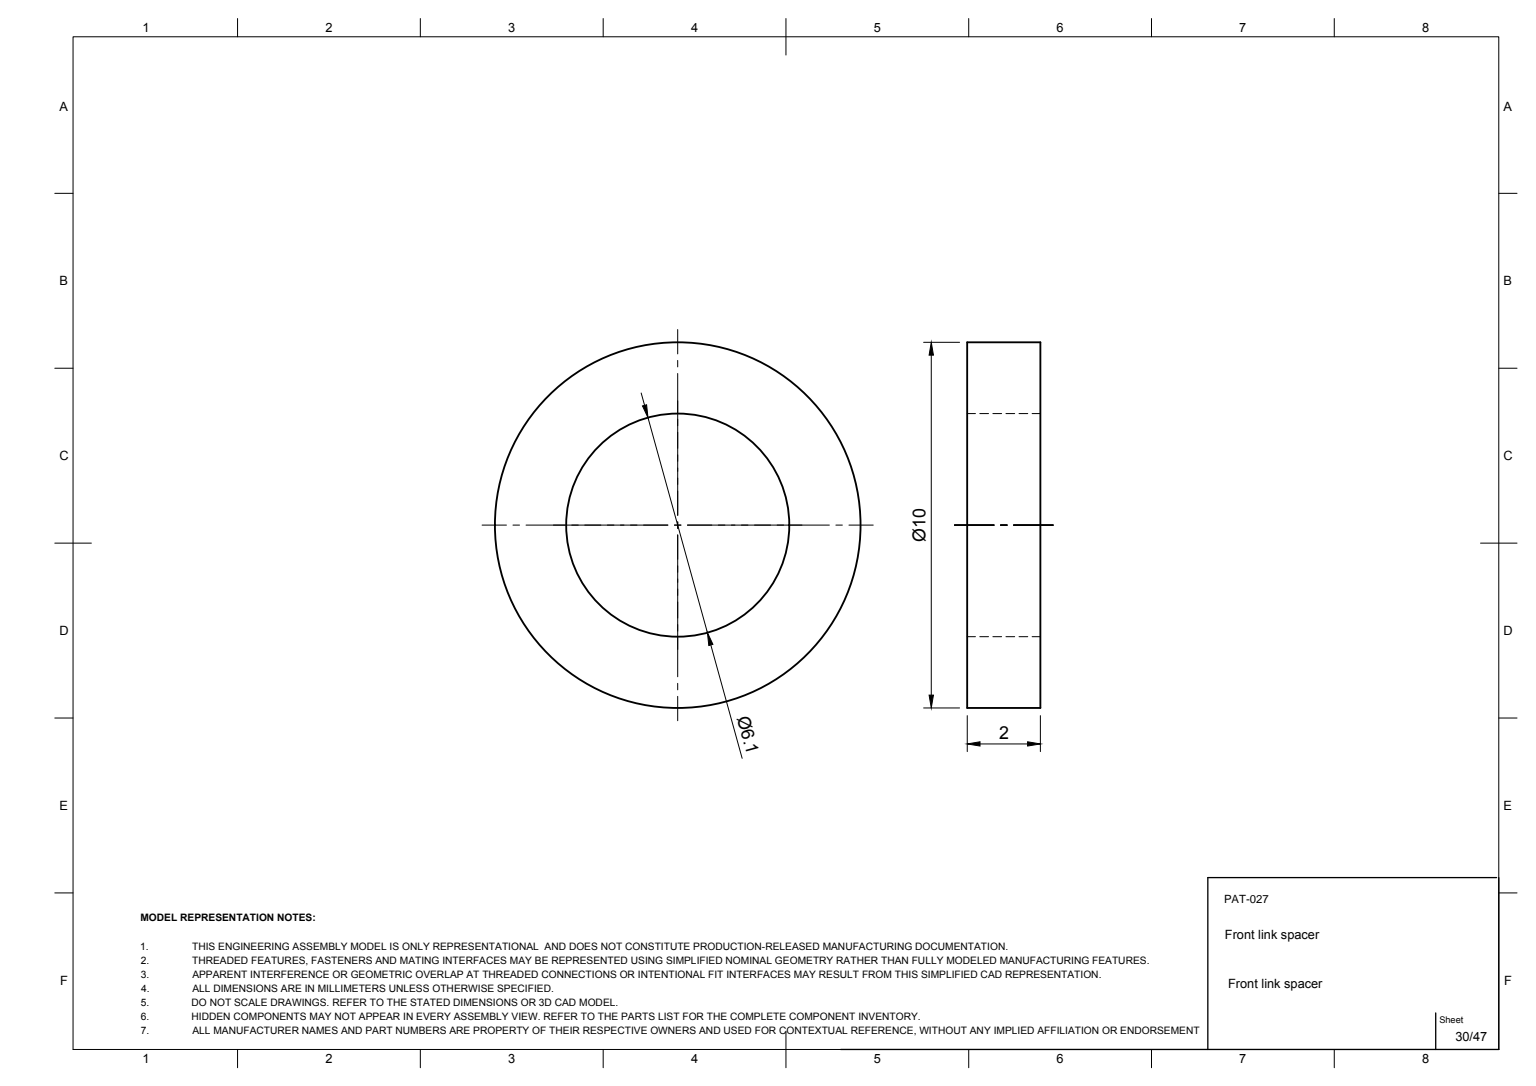
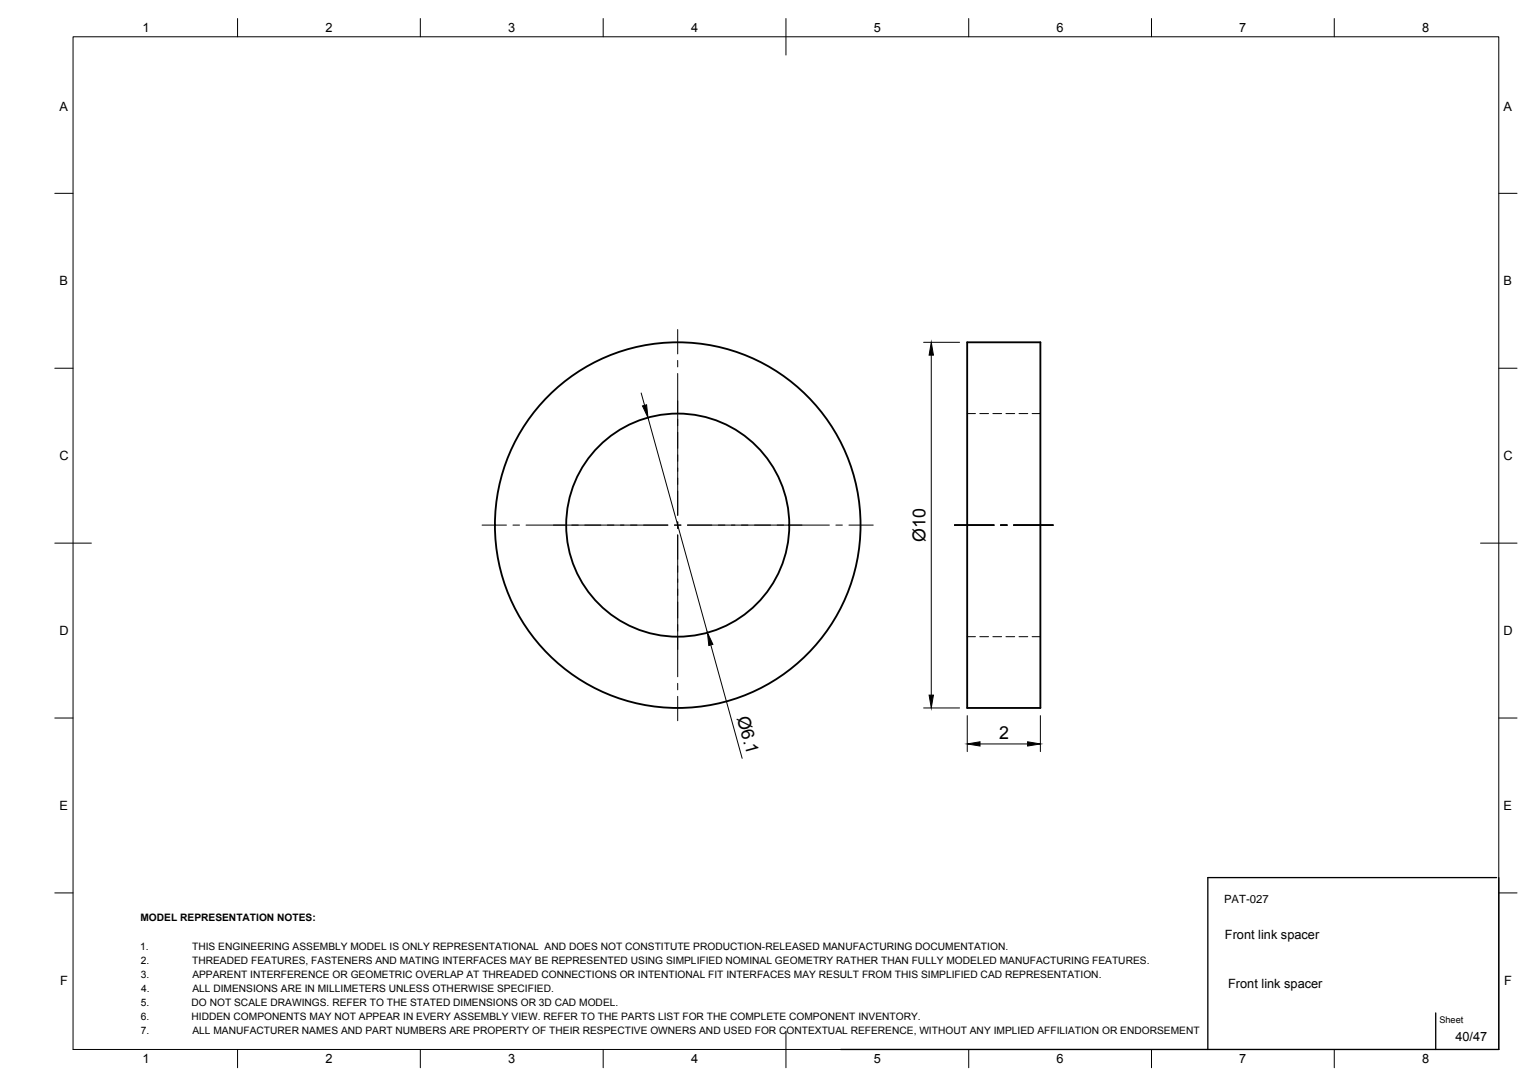
ISO-10303-21;
HEADER;
/* Generated by software containing ST-Developer
 * from STEP Tools, Inc. (www.steptools.com) 
 */

FILE_DESCRIPTION(
/* description */ ('Crank-driven oscillating fan base (mechanism only)'),

/* implementation_level */ '2;1');

FILE_NAME(
/* name */ 'Front link spacer.step',
/* time_stamp */ '2026-10-28T03:25:00-07:00',
/* author */ (''),
/* organization */ (''),
/* preprocessor_version */ 'ST-DEVELOPER v20.2',
/* originating_system */ 'Autodesk Translation Framework v15.17.0.0',
/* authorisation */ '');

FILE_SCHEMA (('AUTOMOTIVE_DESIGN { 1 0 10303 214 3 1 1 }'));
ENDSEC;

DATA;
#10=MECHANICAL_DESIGN_GEOMETRIC_PRESENTATION_REPRESENTATION('',(#467),#11916);
#379=SHAPE_REPRESENTATION_RELATIONSHIP('SRR','None',#12105,#419);
#419=ADVANCED_BREP_SHAPE_REPRESENTATION('',(#514),#11896);
#467=STYLED_ITEM('',(#12361),#514);
#514=MANIFOLD_SOLID_BREP('Body1',#6098);
#642=FACE_BOUND('',#1607,.T.);
#643=FACE_BOUND('',#1609,.T.);
#800=PLANE('',#7087);
#801=PLANE('',#7088);
#1117=FACE_OUTER_BOUND('',#1604,.T.);
#1118=FACE_OUTER_BOUND('',#1605,.T.);
#1119=FACE_OUTER_BOUND('',#1606,.T.);
#1120=FACE_OUTER_BOUND('',#1608,.T.);
#1604=EDGE_LOOP('',(#5012,#5013,#5014,#5015));
#1605=EDGE_LOOP('',(#5016,#5017,#5018,#5019));
#1606=EDGE_LOOP('',(#5020));
#1607=EDGE_LOOP('',(#5021));
#1608=EDGE_LOOP('',(#5022));
#1609=EDGE_LOOP('',(#5023));
#1975=LINE('',#11100,#2308);
#1976=LINE('',#11106,#2309);
#2308=VECTOR('',#8636,0.305);
#2309=VECTOR('',#8643,0.5);
#2723=CIRCLE('',#7082,0.305);
#2724=CIRCLE('',#7083,0.305);
#2725=CIRCLE('',#7085,0.5);
#2726=CIRCLE('',#7086,0.5);
#3154=VERTEX_POINT('',#11097);
#3155=VERTEX_POINT('',#11099);
#3156=VERTEX_POINT('',#11103);
#3157=VERTEX_POINT('',#11105);
#3801=EDGE_CURVE('',#3154,#3154,#2723,.T.);
#3802=EDGE_CURVE('',#3154,#3155,#1975,.T.);
#3803=EDGE_CURVE('',#3155,#3155,#2724,.T.);
#3804=EDGE_CURVE('',#3156,#3156,#2725,.T.);
#3805=EDGE_CURVE('',#3156,#3157,#1976,.T.);
#3806=EDGE_CURVE('',#3157,#3157,#2726,.T.);
#5012=ORIENTED_EDGE('',*,*,#3801,.F.);
#5013=ORIENTED_EDGE('',*,*,#3802,.T.);
#5014=ORIENTED_EDGE('',*,*,#3803,.T.);
#5015=ORIENTED_EDGE('',*,*,#3802,.F.);
#5016=ORIENTED_EDGE('',*,*,#3804,.F.);
#5017=ORIENTED_EDGE('',*,*,#3805,.T.);
#5018=ORIENTED_EDGE('',*,*,#3806,.T.);
#5019=ORIENTED_EDGE('',*,*,#3805,.F.);
#5020=ORIENTED_EDGE('',*,*,#3804,.T.);
#5021=ORIENTED_EDGE('',*,*,#3801,.T.);
#5022=ORIENTED_EDGE('',*,*,#3806,.F.);
#5023=ORIENTED_EDGE('',*,*,#3803,.F.);
#5644=CYLINDRICAL_SURFACE('',#7081,0.305);
#5645=CYLINDRICAL_SURFACE('',#7084,0.5);
#5923=ADVANCED_FACE('',(#1117),#5644,.F.);
#5924=ADVANCED_FACE('',(#1118),#5645,.T.);
#5925=ADVANCED_FACE('',(#1119,#642),#800,.T.);
#5926=ADVANCED_FACE('',(#1120,#643),#801,.F.);
#6098=CLOSED_SHELL('',(#5923,#5924,#5925,#5926));
#7080=AXIS2_PLACEMENT_3D('',#11095,#8630,#8631);
#7081=AXIS2_PLACEMENT_3D('',#11096,#8632,#8633);
#7082=AXIS2_PLACEMENT_3D('',#11098,#8634,#8635);
#7083=AXIS2_PLACEMENT_3D('',#11101,#8637,#8638);
#7084=AXIS2_PLACEMENT_3D('',#11102,#8639,#8640);
#7085=AXIS2_PLACEMENT_3D('',#11104,#8641,#8642);
#7086=AXIS2_PLACEMENT_3D('',#11107,#8644,#8645);
#7087=AXIS2_PLACEMENT_3D('',#11108,#8646,#8647);
#7088=AXIS2_PLACEMENT_3D('',#11109,#8648,#8649);
#8630=DIRECTION('axis',(0.,0.,1.));
#8631=DIRECTION('refdir',(1.,0.,0.));
#8632=DIRECTION('center_axis',(0.,0.,1.));
#8633=DIRECTION('ref_axis',(1.,0.,0.));
#8634=DIRECTION('center_axis',(0.,0.,-1.));
#8635=DIRECTION('ref_axis',(1.,0.,0.));
#8636=DIRECTION('',(0.,0.,-1.));
#8637=DIRECTION('center_axis',(0.,0.,-1.));
#8638=DIRECTION('ref_axis',(1.,0.,0.));
#8639=DIRECTION('center_axis',(0.,0.,1.));
#8640=DIRECTION('ref_axis',(1.,0.,0.));
#8641=DIRECTION('center_axis',(0.,0.,1.));
#8642=DIRECTION('ref_axis',(1.,0.,0.));
#8643=DIRECTION('',(0.,0.,-1.));
#8644=DIRECTION('center_axis',(0.,0.,1.));
#8645=DIRECTION('ref_axis',(1.,0.,0.));
#8646=DIRECTION('center_axis',(0.,0.,1.));
#8647=DIRECTION('ref_axis',(1.,0.,0.));
#8648=DIRECTION('center_axis',(0.,0.,1.));
#8649=DIRECTION('ref_axis',(1.,0.,0.));
#11095=CARTESIAN_POINT('',(0.,0.,0.));
#11096=CARTESIAN_POINT('Origin',(-0.429855350392604,2.61349944954989,9.4));
#11097=CARTESIAN_POINT('',(-0.734855350392604,2.61349944954989,9.6));
#11098=CARTESIAN_POINT('Origin',(-0.429855350392604,2.61349944954989,9.6));
#11099=CARTESIAN_POINT('',(-0.734855350392604,2.61349944954989,9.4));
#11100=CARTESIAN_POINT('',(-0.734855350392604,2.61349944954989,9.4));
#11101=CARTESIAN_POINT('Origin',(-0.429855350392604,2.61349944954989,9.4));
#11102=CARTESIAN_POINT('Origin',(-0.429855350392604,2.61349944954989,9.4));
#11103=CARTESIAN_POINT('',(-0.929855350392604,2.61349944954989,9.6));
#11104=CARTESIAN_POINT('Origin',(-0.429855350392604,2.61349944954989,9.6));
#11105=CARTESIAN_POINT('',(-0.929855350392604,2.61349944954989,9.4));
#11106=CARTESIAN_POINT('',(-0.929855350392604,2.61349944954989,9.4));
#11107=CARTESIAN_POINT('Origin',(-0.429855350392604,2.61349944954989,9.4));
#11108=CARTESIAN_POINT('Origin',(-0.429855350392604,2.61349944954989,9.6));
#11109=CARTESIAN_POINT('Origin',(-0.429855350392604,2.61349944954989,9.4));
#11849=UNCERTAINTY_MEASURE_WITH_UNIT(LENGTH_MEASURE(0.001),#11917,
'DISTANCE_ACCURACY_VALUE',
'Maximum model space distance between geometric entities at asserted c
onnectivities');
#11869=UNCERTAINTY_MEASURE_WITH_UNIT(LENGTH_MEASURE(0.001),#11917,
'DISTANCE_ACCURACY_VALUE',
'Maximum model space distance between geometric entities at asserted c
onnectivities');
#11896=(
GEOMETRIC_REPRESENTATION_CONTEXT(3)
GLOBAL_UNCERTAINTY_ASSIGNED_CONTEXT((#11849))
GLOBAL_UNIT_ASSIGNED_CONTEXT((#11917,#11919,#11920))
REPRESENTATION_CONTEXT('','3D')
);
#11916=(
GEOMETRIC_REPRESENTATION_CONTEXT(3)
GLOBAL_UNCERTAINTY_ASSIGNED_CONTEXT((#11869))
GLOBAL_UNIT_ASSIGNED_CONTEXT((#11917,#11919,#11920))
REPRESENTATION_CONTEXT('','3D')
);
#11917=(
LENGTH_UNIT()
NAMED_UNIT(*)
SI_UNIT(.CENTI.,.METRE.)
);
#11919=(
NAMED_UNIT(*)
PLANE_ANGLE_UNIT()
SI_UNIT($,.RADIAN.)
);
#11920=(
NAMED_UNIT(*)
SI_UNIT($,.STERADIAN.)
SOLID_ANGLE_UNIT()
);
#11947=SHAPE_DEFINITION_REPRESENTATION(#11998,#12105);
#11998=PRODUCT_DEFINITION_SHAPE('',$,#12152);
#12105=SHAPE_REPRESENTATION('',(#7080),#11896);
#12125=PRODUCT_DEFINITION_CONTEXT('part definition',#12265,'design');
#12152=PRODUCT_DEFINITION('Front link spacer','Front link spacer',#12198,
#12125);
#12198=PRODUCT_DEFINITION_FORMATION('',$,#12293);
#12265=APPLICATION_CONTEXT(
'Core Data for Automotive Mechanical Design Process');
#12266=PRODUCT_CONTEXT('part definition',#12265,'mechanical');
#12293=PRODUCT('Front link spacer','Front link spacer',
'Front link spacer',(#12266));
#12355=COLOUR_RGB('Light Blue',0.38,0.62,0.78);
#12356=FILL_AREA_STYLE_COLOUR('',#12355);
#12357=FILL_AREA_STYLE('',(#12356));
#12358=SURFACE_STYLE_FILL_AREA(#12357);
#12359=SURFACE_SIDE_STYLE('',(#12358));
#12360=SURFACE_STYLE_USAGE(.BOTH.,#12359);
#12361=PRESENTATION_STYLE_ASSIGNMENT((#12360));
ENDSEC;
END-ISO-10303-21;
